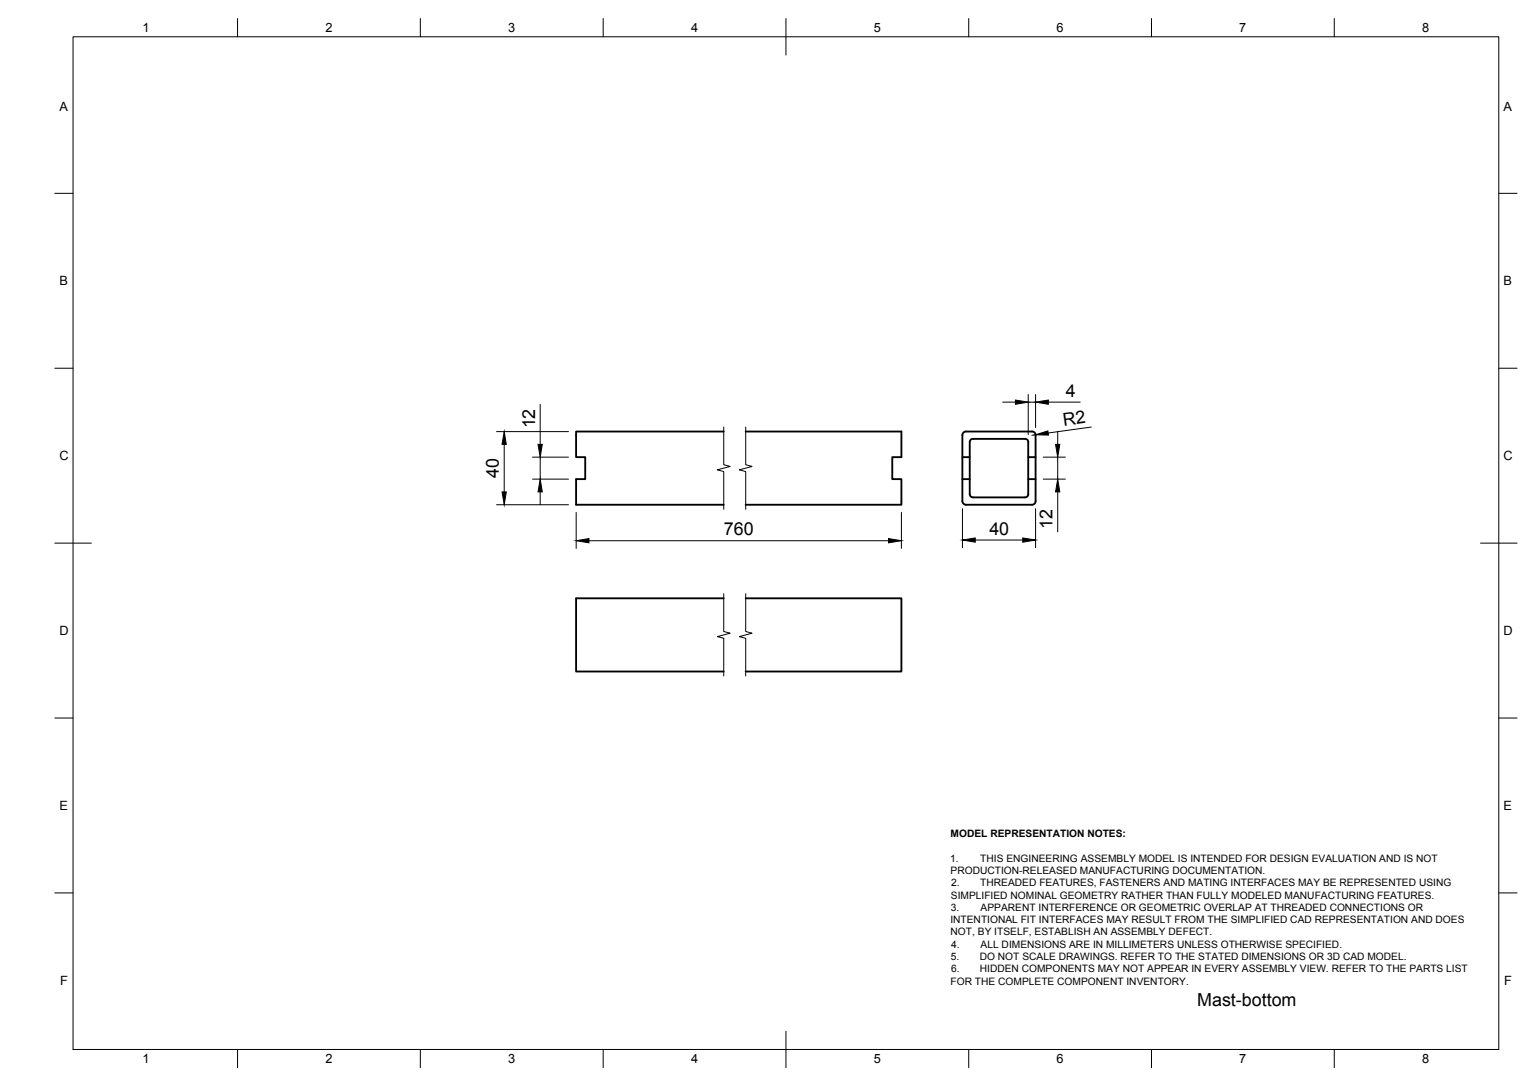
ISO-10303-21;
HEADER;
/* Generated by software containing ST-Developer
 * from STEP Tools, Inc. (www.steptools.com) 
 */

FILE_DESCRIPTION(
/* description */ (''),
/* implementation_level */ '2;1');

FILE_NAME(
/* name */ 'Mast-bottom.step',
/* time_stamp */ '2026-10-07T11:02:43-07:00',
/* author */ (''),
/* organization */ (''),
/* preprocessor_version */ 'ST-DEVELOPER v20.2',
/* originating_system */ 'Autodesk Translation Framework v15.15.0.0',
/* authorisation */ '');

FILE_SCHEMA (('AUTOMOTIVE_DESIGN { 1 0 10303 214 3 1 1 }'));
ENDSEC;

DATA;
#10=MECHANICAL_DESIGN_GEOMETRIC_PRESENTATION_REPRESENTATION('',(#66),#5505);
#52=SHAPE_REPRESENTATION_RELATIONSHIP('SRR','None',#5537,#59);
#59=ADVANCED_BREP_SHAPE_REPRESENTATION('',(#73),#5498);
#66=STYLED_ITEM('',(#5581),#73);
#73=MANIFOLD_SOLID_BREP('Body1',#3293);
#80=FACE_BOUND('',#416,.T.);
#81=FACE_BOUND('',#417,.T.);
#82=FACE_BOUND('',#428,.T.);
#83=FACE_BOUND('',#429,.T.);
#113=CYLINDRICAL_SURFACE('',#3399,2.);
#114=CYLINDRICAL_SURFACE('',#3401,2.);
#115=CYLINDRICAL_SURFACE('',#3404,2.);
#116=CYLINDRICAL_SURFACE('',#3406,2.);
#117=CYLINDRICAL_SURFACE('',#3414,1.8);
#118=CYLINDRICAL_SURFACE('',#3415,1.8);
#119=CYLINDRICAL_SURFACE('',#3417,1.8);
#120=CYLINDRICAL_SURFACE('',#3418,1.8);
#153=CIRCLE('',#3385,1.8);
#154=CIRCLE('',#3386,1.8);
#155=CIRCLE('',#3387,2.);
#156=CIRCLE('',#3388,2.);
#157=CIRCLE('',#3392,2.);
#158=CIRCLE('',#3393,2.);
#159=CIRCLE('',#3394,1.8);
#160=CIRCLE('',#3395,1.8);
#161=CIRCLE('',#3400,2.);
#162=CIRCLE('',#3402,2.);
#163=CIRCLE('',#3405,2.);
#164=CIRCLE('',#3407,2.);
#165=CIRCLE('',#3409,1.8);
#166=CIRCLE('',#3410,1.8);
#167=CIRCLE('',#3412,1.8);
#168=CIRCLE('',#3413,1.8);
#236=FACE_OUTER_BOUND('',#402,.T.);
#237=FACE_OUTER_BOUND('',#403,.T.);
#238=FACE_OUTER_BOUND('',#404,.T.);
#239=FACE_OUTER_BOUND('',#405,.T.);
#240=FACE_OUTER_BOUND('',#406,.T.);
#241=FACE_OUTER_BOUND('',#407,.T.);
#242=FACE_OUTER_BOUND('',#408,.T.);
#243=FACE_OUTER_BOUND('',#409,.T.);
#244=FACE_OUTER_BOUND('',#410,.T.);
#245=FACE_OUTER_BOUND('',#411,.T.);
#246=FACE_OUTER_BOUND('',#412,.T.);
#247=FACE_OUTER_BOUND('',#413,.T.);
#248=FACE_OUTER_BOUND('',#414,.T.);
#249=FACE_OUTER_BOUND('',#415,.T.);
#250=FACE_OUTER_BOUND('',#418,.T.);
#251=FACE_OUTER_BOUND('',#419,.T.);
#252=FACE_OUTER_BOUND('',#420,.T.);
#253=FACE_OUTER_BOUND('',#421,.T.);
#254=FACE_OUTER_BOUND('',#422,.T.);
#255=FACE_OUTER_BOUND('',#423,.T.);
#256=FACE_OUTER_BOUND('',#424,.T.);
#257=FACE_OUTER_BOUND('',#425,.T.);
#258=FACE_OUTER_BOUND('',#426,.T.);
#259=FACE_OUTER_BOUND('',#427,.T.);
#260=FACE_OUTER_BOUND('',#430,.T.);
#261=FACE_OUTER_BOUND('',#431,.T.);
#262=FACE_OUTER_BOUND('',#432,.T.);
#263=FACE_OUTER_BOUND('',#433,.T.);
#264=FACE_OUTER_BOUND('',#434,.T.);
#265=FACE_OUTER_BOUND('',#435,.T.);
#266=FACE_OUTER_BOUND('',#436,.T.);
#267=FACE_OUTER_BOUND('',#437,.T.);
#268=FACE_OUTER_BOUND('',#438,.T.);
#269=FACE_OUTER_BOUND('',#439,.T.);
#270=FACE_OUTER_BOUND('',#440,.T.);
#271=FACE_OUTER_BOUND('',#441,.T.);
#272=FACE_OUTER_BOUND('',#442,.T.);
#273=FACE_OUTER_BOUND('',#443,.T.);
#274=FACE_OUTER_BOUND('',#444,.T.);
#275=FACE_OUTER_BOUND('',#445,.T.);
#402=EDGE_LOOP('',(#2096,#2097,#2098,#2099));
#403=EDGE_LOOP('',(#2100,#2101,#2102,#2103));
#404=EDGE_LOOP('',(#2104,#2105,#2106,#2107));
#405=EDGE_LOOP('',(#2108,#2109,#2110,#2111));
#406=EDGE_LOOP('',(#2112,#2113,#2114,#2115,#2116,#2117,#2118,#2119,#2120,
#2121,#2122,#2123));
#407=EDGE_LOOP('',(#2124,#2125,#2126,#2127,#2128,#2129,#2130,#2131,#2132,
#2133,#2134,#2135));
#408=EDGE_LOOP('',(#2136,#2137,#2138,#2139,#2140,#2141,#2142,#2143,#2144,
#2145,#2146,#2147));
#409=EDGE_LOOP('',(#2148,#2149,#2150,#2151,#2152,#2153,#2154,#2155,#2156,
#2157,#2158,#2159));
#410=EDGE_LOOP('',(#2160,#2161,#2162,#2163,#2164,#2165,#2166,#2167,#2168,
#2169,#2170,#2171));
#411=EDGE_LOOP('',(#2172,#2173,#2174,#2175,#2176,#2177,#2178,#2179,#2180,
#2181,#2182,#2183));
#412=EDGE_LOOP('',(#2184,#2185,#2186,#2187));
#413=EDGE_LOOP('',(#2188,#2189,#2190,#2191));
#414=EDGE_LOOP('',(#2192,#2193,#2194,#2195));
#415=EDGE_LOOP('',(#2196,#2197,#2198,#2199));
#416=EDGE_LOOP('',(#2200,#2201,#2202,#2203));
#417=EDGE_LOOP('',(#2204,#2205,#2206,#2207));
#418=EDGE_LOOP('',(#2208,#2209,#2210,#2211));
#419=EDGE_LOOP('',(#2212,#2213,#2214,#2215));
#420=EDGE_LOOP('',(#2216,#2217,#2218,#2219,#2220,#2221,#2222,#2223,#2224,
#2225,#2226,#2227));
#421=EDGE_LOOP('',(#2228,#2229,#2230,#2231,#2232,#2233,#2234,#2235,#2236,
#2237,#2238,#2239));
#422=EDGE_LOOP('',(#2240,#2241,#2242,#2243));
#423=EDGE_LOOP('',(#2244,#2245,#2246,#2247));
#424=EDGE_LOOP('',(#2248,#2249,#2250,#2251));
#425=EDGE_LOOP('',(#2252,#2253,#2254,#2255));
#426=EDGE_LOOP('',(#2256,#2257,#2258,#2259));
#427=EDGE_LOOP('',(#2260,#2261,#2262,#2263));
#428=EDGE_LOOP('',(#2264,#2265,#2266,#2267));
#429=EDGE_LOOP('',(#2268,#2269,#2270,#2271));
#430=EDGE_LOOP('',(#2272,#2273,#2274,#2275));
#431=EDGE_LOOP('',(#2276,#2277,#2278,#2279));
#432=EDGE_LOOP('',(#2280,#2281,#2282,#2283));
#433=EDGE_LOOP('',(#2284,#2285,#2286,#2287));
#434=EDGE_LOOP('',(#2288,#2289,#2290,#2291));
#435=EDGE_LOOP('',(#2292,#2293,#2294,#2295));
#436=EDGE_LOOP('',(#2296,#2297,#2298,#2299));
#437=EDGE_LOOP('',(#2300,#2301,#2302,#2303));
#438=EDGE_LOOP('',(#2304,#2305,#2306,#2307));
#439=EDGE_LOOP('',(#2308,#2309,#2310,#2311));
#440=EDGE_LOOP('',(#2312,#2313,#2314,#2315));
#441=EDGE_LOOP('',(#2316,#2317,#2318,#2319));
#442=EDGE_LOOP('',(#2320,#2321,#2322,#2323));
#443=EDGE_LOOP('',(#2324,#2325,#2326,#2327));
#444=EDGE_LOOP('',(#2328,#2329,#2330,#2331));
#445=EDGE_LOOP('',(#2332,#2333,#2334,#2335));
#601=LINE('',#4554,#971);
#602=LINE('',#4556,#972);
#603=LINE('',#4558,#973);
#604=LINE('',#4559,#974);
#605=LINE('',#4562,#975);
#606=LINE('',#4564,#976);
#607=LINE('',#4565,#977);
#608=LINE('',#4568,#978);
#609=LINE('',#4570,#979);
#610=LINE('',#4571,#980);
#611=LINE('',#4573,#981);
#612=LINE('',#4574,#982);
#613=LINE('',#4578,#983);
#614=LINE('',#4580,#984);
#615=LINE('',#4582,#985);
#616=LINE('',#4586,#986);
#617=LINE('',#4590,#987);
#618=LINE('',#4592,#988);
#619=LINE('',#4594,#989);
#620=LINE('',#4598,#990);
#621=LINE('',#4603,#991);
#622=LINE('',#4605,#992);
#623=LINE('',#4606,#993);
#624=LINE('',#4608,#994);
#625=LINE('',#4610,#995);
#626=LINE('',#4612,#996);
#627=LINE('',#4614,#997);
#628=LINE('',#4616,#998);
#629=LINE('',#4618,#999);
#630=LINE('',#4620,#1000);
#631=LINE('',#4621,#1001);
#632=LINE('',#4625,#1002);
#633=LINE('',#4627,#1003);
#634=LINE('',#4629,#1004);
#635=LINE('',#4631,#1005);
#636=LINE('',#4633,#1006);
#637=LINE('',#4635,#1007);
#638=LINE('',#4637,#1008);
#639=LINE('',#4639,#1009);
#640=LINE('',#4640,#1010);
#641=LINE('',#4642,#1011);
#642=LINE('',#4643,#1012);
#643=LINE('',#4646,#1013);
#644=LINE('',#4648,#1014);
#645=LINE('',#4652,#1015);
#646=LINE('',#4656,#1016);
#647=LINE('',#4657,#1017);
#648=LINE('',#4661,#1018);
#649=LINE('',#4666,#1019);
#650=LINE('',#4668,#1020);
#651=LINE('',#4669,#1021);
#652=LINE('',#4671,#1022);
#653=LINE('',#4673,#1023);
#654=LINE('',#4675,#1024);
#655=LINE('',#4677,#1025);
#656=LINE('',#4678,#1026);
#657=LINE('',#4680,#1027);
#658=LINE('',#4681,#1028);
#659=LINE('',#4685,#1029);
#660=LINE('',#4687,#1030);
#661=LINE('',#4688,#1031);
#662=LINE('',#4690,#1032);
#663=LINE('',#4692,#1033);
#664=LINE('',#4694,#1034);
#665=LINE('',#4696,#1035);
#666=LINE('',#4697,#1036);
#667=LINE('',#4699,#1037);
#668=LINE('',#4700,#1038);
#669=LINE('',#4704,#1039);
#670=LINE('',#4705,#1040);
#671=LINE('',#4706,#1041);
#672=LINE('',#4711,#1042);
#673=LINE('',#4715,#1043);
#674=LINE('',#4716,#1044);
#675=LINE('',#4719,#1045);
#676=LINE('',#4721,#1046);
#677=LINE('',#4723,#1047);
#678=LINE('',#4724,#1048);
#679=LINE('',#4730,#1049);
#680=LINE('',#4731,#1050);
#681=LINE('',#4735,#1051);
#682=LINE('',#4738,#1052);
#683=LINE('',#4742,#1053);
#684=LINE('',#4744,#1054);
#685=LINE('',#4746,#1055);
#686=LINE('',#4748,#1056);
#687=LINE('',#4750,#1057);
#688=LINE('',#4753,#1058);
#689=LINE('',#4757,#1059);
#690=LINE('',#4759,#1060);
#691=LINE('',#4761,#1061);
#692=LINE('',#4762,#1062);
#693=LINE('',#4764,#1063);
#694=LINE('',#4766,#1064);
#695=LINE('',#4769,#1065);
#696=LINE('',#4771,#1066);
#697=LINE('',#4774,#1067);
#698=LINE('',#4776,#1068);
#699=LINE('',#4779,#1069);
#700=LINE('',#4781,#1070);
#701=LINE('',#4784,#1071);
#702=LINE('',#4785,#1072);
#703=LINE('',#4787,#1073);
#704=LINE('',#4789,#1074);
#971=VECTOR('',#3651,1000.);
#972=VECTOR('',#3652,1000.);
#973=VECTOR('',#3653,1000.);
#974=VECTOR('',#3654,1000.);
#975=VECTOR('',#3657,1000.);
#976=VECTOR('',#3658,1000.);
#977=VECTOR('',#3659,1000.);
#978=VECTOR('',#3662,1000.);
#979=VECTOR('',#3663,1000.);
#980=VECTOR('',#3664,1000.);
#981=VECTOR('',#3667,1000.);
#982=VECTOR('',#3668,1000.);
#983=VECTOR('',#3671,1000.);
#984=VECTOR('',#3672,1000.);
#985=VECTOR('',#3673,1000.);
#986=VECTOR('',#3676,1000.);
#987=VECTOR('',#3679,1000.);
#988=VECTOR('',#3680,1000.);
#989=VECTOR('',#3681,1000.);
#990=VECTOR('',#3684,1000.);
#991=VECTOR('',#3689,1000.);
#992=VECTOR('',#3690,1000.);
#993=VECTOR('',#3691,1000.);
#994=VECTOR('',#3692,1000.);
#995=VECTOR('',#3693,1000.);
#996=VECTOR('',#3694,1000.);
#997=VECTOR('',#3695,1000.);
#998=VECTOR('',#3696,1000.);
#999=VECTOR('',#3697,1000.);
#1000=VECTOR('',#3698,1000.);
#1001=VECTOR('',#3699,1000.);
#1002=VECTOR('',#3702,1000.);
#1003=VECTOR('',#3703,1000.);
#1004=VECTOR('',#3704,1000.);
#1005=VECTOR('',#3705,1000.);
#1006=VECTOR('',#3706,1000.);
#1007=VECTOR('',#3707,1000.);
#1008=VECTOR('',#3708,1000.);
#1009=VECTOR('',#3709,1000.);
#1010=VECTOR('',#3710,1000.);
#1011=VECTOR('',#3711,1000.);
#1012=VECTOR('',#3712,1000.);
#1013=VECTOR('',#3715,1000.);
#1014=VECTOR('',#3716,1000.);
#1015=VECTOR('',#3719,1000.);
#1016=VECTOR('',#3722,1000.);
#1017=VECTOR('',#3723,1000.);
#1018=VECTOR('',#3726,1000.);
#1019=VECTOR('',#3731,1000.);
#1020=VECTOR('',#3732,1000.);
#1021=VECTOR('',#3733,1000.);
#1022=VECTOR('',#3734,1000.);
#1023=VECTOR('',#3735,1000.);
#1024=VECTOR('',#3736,1000.);
#1025=VECTOR('',#3737,1000.);
#1026=VECTOR('',#3738,1000.);
#1027=VECTOR('',#3739,1000.);
#1028=VECTOR('',#3740,1000.);
#1029=VECTOR('',#3743,1000.);
#1030=VECTOR('',#3744,1000.);
#1031=VECTOR('',#3745,1000.);
#1032=VECTOR('',#3746,1000.);
#1033=VECTOR('',#3747,1000.);
#1034=VECTOR('',#3748,1000.);
#1035=VECTOR('',#3749,1000.);
#1036=VECTOR('',#3750,1000.);
#1037=VECTOR('',#3751,1000.);
#1038=VECTOR('',#3752,1000.);
#1039=VECTOR('',#3755,1000.);
#1040=VECTOR('',#3756,1000.);
#1041=VECTOR('',#3757,1000.);
#1042=VECTOR('',#3764,1000.);
#1043=VECTOR('',#3769,1000.);
#1044=VECTOR('',#3770,1000.);
#1045=VECTOR('',#3771,1000.);
#1046=VECTOR('',#3772,1000.);
#1047=VECTOR('',#3773,1000.);
#1048=VECTOR('',#3774,1000.);
#1049=VECTOR('',#3785,1000.);
#1050=VECTOR('',#3786,1000.);
#1051=VECTOR('',#3789,1000.);
#1052=VECTOR('',#3794,1000.);
#1053=VECTOR('',#3797,1000.);
#1054=VECTOR('',#3800,1000.);
#1055=VECTOR('',#3803,1000.);
#1056=VECTOR('',#3806,1000.);
#1057=VECTOR('',#3809,1000.);
#1058=VECTOR('',#3814,1000.);
#1059=VECTOR('',#3817,1000.);
#1060=VECTOR('',#3818,1000.);
#1061=VECTOR('',#3819,1000.);
#1062=VECTOR('',#3820,1000.);
#1063=VECTOR('',#3823,1000.);
#1064=VECTOR('',#3826,1000.);
#1065=VECTOR('',#3831,1000.);
#1066=VECTOR('',#3834,1000.);
#1067=VECTOR('',#3839,1000.);
#1068=VECTOR('',#3842,1000.);
#1069=VECTOR('',#3847,1000.);
#1070=VECTOR('',#3850,1000.);
#1071=VECTOR('',#3855,1000.);
#1072=VECTOR('',#3856,1000.);
#1073=VECTOR('',#3859,1000.);
#1074=VECTOR('',#3862,1000.);
#1341=VERTEX_POINT('',#4552);
#1342=VERTEX_POINT('',#4553);
#1343=VERTEX_POINT('',#4555);
#1344=VERTEX_POINT('',#4557);
#1345=VERTEX_POINT('',#4561);
#1346=VERTEX_POINT('',#4563);
#1347=VERTEX_POINT('',#4567);
#1348=VERTEX_POINT('',#4569);
#1349=VERTEX_POINT('',#4576);
#1350=VERTEX_POINT('',#4577);
#1351=VERTEX_POINT('',#4579);
#1352=VERTEX_POINT('',#4581);
#1353=VERTEX_POINT('',#4583);
#1354=VERTEX_POINT('',#4585);
#1355=VERTEX_POINT('',#4587);
#1356=VERTEX_POINT('',#4589);
#1357=VERTEX_POINT('',#4591);
#1358=VERTEX_POINT('',#4593);
#1359=VERTEX_POINT('',#4595);
#1360=VERTEX_POINT('',#4597);
#1361=VERTEX_POINT('',#4601);
#1362=VERTEX_POINT('',#4602);
#1363=VERTEX_POINT('',#4604);
#1364=VERTEX_POINT('',#4607);
#1365=VERTEX_POINT('',#4609);
#1366=VERTEX_POINT('',#4611);
#1367=VERTEX_POINT('',#4613);
#1368=VERTEX_POINT('',#4615);
#1369=VERTEX_POINT('',#4617);
#1370=VERTEX_POINT('',#4619);
#1371=VERTEX_POINT('',#4623);
#1372=VERTEX_POINT('',#4624);
#1373=VERTEX_POINT('',#4626);
#1374=VERTEX_POINT('',#4628);
#1375=VERTEX_POINT('',#4630);
#1376=VERTEX_POINT('',#4632);
#1377=VERTEX_POINT('',#4634);
#1378=VERTEX_POINT('',#4636);
#1379=VERTEX_POINT('',#4638);
#1380=VERTEX_POINT('',#4641);
#1381=VERTEX_POINT('',#4645);
#1382=VERTEX_POINT('',#4647);
#1383=VERTEX_POINT('',#4649);
#1384=VERTEX_POINT('',#4651);
#1385=VERTEX_POINT('',#4653);
#1386=VERTEX_POINT('',#4655);
#1387=VERTEX_POINT('',#4658);
#1388=VERTEX_POINT('',#4660);
#1389=VERTEX_POINT('',#4664);
#1390=VERTEX_POINT('',#4665);
#1391=VERTEX_POINT('',#4667);
#1392=VERTEX_POINT('',#4670);
#1393=VERTEX_POINT('',#4672);
#1394=VERTEX_POINT('',#4674);
#1395=VERTEX_POINT('',#4676);
#1396=VERTEX_POINT('',#4679);
#1397=VERTEX_POINT('',#4683);
#1398=VERTEX_POINT('',#4684);
#1399=VERTEX_POINT('',#4686);
#1400=VERTEX_POINT('',#4689);
#1401=VERTEX_POINT('',#4691);
#1402=VERTEX_POINT('',#4693);
#1403=VERTEX_POINT('',#4695);
#1404=VERTEX_POINT('',#4698);
#1405=VERTEX_POINT('',#4702);
#1406=VERTEX_POINT('',#4703);
#1407=VERTEX_POINT('',#4710);
#1408=VERTEX_POINT('',#4714);
#1409=VERTEX_POINT('',#4717);
#1410=VERTEX_POINT('',#4718);
#1411=VERTEX_POINT('',#4720);
#1412=VERTEX_POINT('',#4722);
#1413=VERTEX_POINT('',#4732);
#1414=VERTEX_POINT('',#4734);
#1415=VERTEX_POINT('',#4739);
#1416=VERTEX_POINT('',#4741);
#1417=VERTEX_POINT('',#4755);
#1418=VERTEX_POINT('',#4756);
#1419=VERTEX_POINT('',#4758);
#1420=VERTEX_POINT('',#4760);
#1643=EDGE_CURVE('',#1341,#1342,#601,.T.);
#1644=EDGE_CURVE('',#1341,#1343,#602,.T.);
#1645=EDGE_CURVE('',#1343,#1344,#603,.T.);
#1646=EDGE_CURVE('',#1344,#1342,#604,.T.);
#1647=EDGE_CURVE('',#1343,#1345,#605,.T.);
#1648=EDGE_CURVE('',#1345,#1346,#606,.T.);
#1649=EDGE_CURVE('',#1346,#1344,#607,.T.);
#1650=EDGE_CURVE('',#1347,#1345,#608,.T.);
#1651=EDGE_CURVE('',#1347,#1348,#609,.T.);
#1652=EDGE_CURVE('',#1346,#1348,#610,.T.);
#1653=EDGE_CURVE('',#1341,#1347,#611,.T.);
#1654=EDGE_CURVE('',#1348,#1342,#612,.T.);
#1655=EDGE_CURVE('',#1349,#1350,#613,.T.);
#1656=EDGE_CURVE('',#1350,#1351,#614,.T.);
#1657=EDGE_CURVE('',#1351,#1352,#615,.T.);
#1658=EDGE_CURVE('',#1353,#1352,#153,.T.);
#1659=EDGE_CURVE('',#1353,#1354,#616,.T.);
#1660=EDGE_CURVE('',#1355,#1354,#154,.T.);
#1661=EDGE_CURVE('',#1356,#1355,#617,.T.);
#1662=EDGE_CURVE('',#1356,#1357,#618,.T.);
#1663=EDGE_CURVE('',#1357,#1358,#619,.T.);
#1664=EDGE_CURVE('',#1358,#1359,#155,.T.);
#1665=EDGE_CURVE('',#1359,#1360,#620,.T.);
#1666=EDGE_CURVE('',#1360,#1349,#156,.T.);
#1667=EDGE_CURVE('',#1361,#1362,#621,.T.);
#1668=EDGE_CURVE('',#1363,#1361,#622,.T.);
#1669=EDGE_CURVE('',#1363,#1356,#623,.T.);
#1670=EDGE_CURVE('',#1364,#1355,#624,.T.);
#1671=EDGE_CURVE('',#1365,#1364,#625,.F.);
#1672=EDGE_CURVE('',#1366,#1365,#626,.T.);
#1673=EDGE_CURVE('',#1366,#1367,#627,.T.);
#1674=EDGE_CURVE('',#1367,#1368,#628,.T.);
#1675=EDGE_CURVE('',#1369,#1368,#629,.F.);
#1676=EDGE_CURVE('',#1369,#1370,#630,.T.);
#1677=EDGE_CURVE('',#1370,#1362,#631,.T.);
#1678=EDGE_CURVE('',#1371,#1372,#632,.T.);
#1679=EDGE_CURVE('',#1373,#1371,#633,.T.);
#1680=EDGE_CURVE('',#1374,#1373,#634,.T.);
#1681=EDGE_CURVE('',#1374,#1375,#635,.F.);
#1682=EDGE_CURVE('',#1375,#1376,#636,.T.);
#1683=EDGE_CURVE('',#1376,#1377,#637,.T.);
#1684=EDGE_CURVE('',#1378,#1377,#638,.T.);
#1685=EDGE_CURVE('',#1378,#1379,#639,.F.);
#1686=EDGE_CURVE('',#1379,#1352,#640,.T.);
#1687=EDGE_CURVE('',#1351,#1380,#641,.T.);
#1688=EDGE_CURVE('',#1372,#1380,#642,.T.);
#1689=EDGE_CURVE('',#1381,#1368,#643,.F.);
#1690=EDGE_CURVE('',#1382,#1381,#644,.F.);
#1691=EDGE_CURVE('',#1383,#1382,#157,.F.);
#1692=EDGE_CURVE('',#1384,#1383,#645,.F.);
#1693=EDGE_CURVE('',#1385,#1384,#158,.F.);
#1694=EDGE_CURVE('',#1386,#1385,#646,.F.);
#1695=EDGE_CURVE('',#1375,#1386,#647,.F.);
#1696=EDGE_CURVE('',#1374,#1387,#159,.F.);
#1697=EDGE_CURVE('',#1387,#1388,#648,.F.);
#1698=EDGE_CURVE('',#1388,#1369,#160,.F.);
#1699=EDGE_CURVE('',#1389,#1390,#649,.T.);
#1700=EDGE_CURVE('',#1391,#1389,#650,.T.);
#1701=EDGE_CURVE('',#1382,#1391,#651,.T.);
#1702=EDGE_CURVE('',#1381,#1392,#652,.T.);
#1703=EDGE_CURVE('',#1392,#1393,#653,.T.);
#1704=EDGE_CURVE('',#1394,#1393,#654,.T.);
#1705=EDGE_CURVE('',#1394,#1395,#655,.F.);
#1706=EDGE_CURVE('',#1395,#1358,#656,.T.);
#1707=EDGE_CURVE('',#1357,#1396,#657,.T.);
#1708=EDGE_CURVE('',#1390,#1396,#658,.T.);
#1709=EDGE_CURVE('',#1397,#1398,#659,.T.);
#1710=EDGE_CURVE('',#1399,#1397,#660,.T.);
#1711=EDGE_CURVE('',#1399,#1350,#661,.T.);
#1712=EDGE_CURVE('',#1400,#1349,#662,.T.);
#1713=EDGE_CURVE('',#1400,#1401,#663,.F.);
#1714=EDGE_CURVE('',#1402,#1401,#664,.T.);
#1715=EDGE_CURVE('',#1402,#1403,#665,.T.);
#1716=EDGE_CURVE('',#1403,#1386,#666,.T.);
#1717=EDGE_CURVE('',#1385,#1404,#667,.T.);
#1718=EDGE_CURVE('',#1398,#1404,#668,.T.);
#1719=EDGE_CURVE('',#1405,#1406,#669,.T.);
#1720=EDGE_CURVE('',#1384,#1405,#670,.T.);
#1721=EDGE_CURVE('',#1383,#1406,#671,.T.);
#1722=EDGE_CURVE('',#1404,#1405,#161,.T.);
#1723=EDGE_CURVE('',#1407,#1360,#672,.T.);
#1724=EDGE_CURVE('',#1407,#1400,#162,.F.);
#1725=EDGE_CURVE('',#1408,#1359,#673,.T.);
#1726=EDGE_CURVE('',#1408,#1407,#674,.F.);
#1727=EDGE_CURVE('',#1409,#1410,#675,.T.);
#1728=EDGE_CURVE('',#1409,#1411,#676,.T.);
#1729=EDGE_CURVE('',#1411,#1412,#677,.T.);
#1730=EDGE_CURVE('',#1410,#1412,#678,.T.);
#1731=EDGE_CURVE('',#1395,#1408,#163,.F.);
#1732=EDGE_CURVE('',#1406,#1391,#164,.T.);
#1733=EDGE_CURVE('',#1398,#1371,#679,.T.);
#1734=EDGE_CURVE('',#1362,#1389,#680,.T.);
#1735=EDGE_CURVE('',#1413,#1370,#165,.T.);
#1736=EDGE_CURVE('',#1414,#1413,#681,.T.);
#1737=EDGE_CURVE('',#1373,#1414,#166,.T.);
#1738=EDGE_CURVE('',#1394,#1365,#682,.F.);
#1739=EDGE_CURVE('',#1364,#1415,#167,.F.);
#1740=EDGE_CURVE('',#1416,#1415,#683,.F.);
#1741=EDGE_CURVE('',#1416,#1379,#168,.F.);
#1742=EDGE_CURVE('',#1378,#1401,#684,.F.);
#1743=EDGE_CURVE('',#1416,#1353,#685,.T.);
#1744=EDGE_CURVE('',#1387,#1414,#686,.T.);
#1745=EDGE_CURVE('',#1388,#1413,#687,.T.);
#1746=EDGE_CURVE('',#1415,#1354,#688,.T.);
#1747=EDGE_CURVE('',#1417,#1418,#689,.T.);
#1748=EDGE_CURVE('',#1419,#1417,#690,.T.);
#1749=EDGE_CURVE('',#1419,#1420,#691,.T.);
#1750=EDGE_CURVE('',#1420,#1418,#692,.T.);
#1751=EDGE_CURVE('',#1377,#1402,#693,.T.);
#1752=EDGE_CURVE('',#1376,#1403,#694,.T.);
#1753=EDGE_CURVE('',#1392,#1367,#695,.T.);
#1754=EDGE_CURVE('',#1393,#1366,#696,.T.);
#1755=EDGE_CURVE('',#1390,#1361,#697,.T.);
#1756=EDGE_CURVE('',#1396,#1363,#698,.T.);
#1757=EDGE_CURVE('',#1372,#1397,#699,.T.);
#1758=EDGE_CURVE('',#1380,#1399,#700,.T.);
#1759=EDGE_CURVE('',#1418,#1409,#701,.T.);
#1760=EDGE_CURVE('',#1417,#1410,#702,.T.);
#1761=EDGE_CURVE('',#1419,#1412,#703,.T.);
#1762=EDGE_CURVE('',#1420,#1411,#704,.T.);
#2096=ORIENTED_EDGE('',*,*,#1643,.F.);
#2097=ORIENTED_EDGE('',*,*,#1644,.T.);
#2098=ORIENTED_EDGE('',*,*,#1645,.T.);
#2099=ORIENTED_EDGE('',*,*,#1646,.T.);
#2100=ORIENTED_EDGE('',*,*,#1645,.F.);
#2101=ORIENTED_EDGE('',*,*,#1647,.T.);
#2102=ORIENTED_EDGE('',*,*,#1648,.T.);
#2103=ORIENTED_EDGE('',*,*,#1649,.T.);
#2104=ORIENTED_EDGE('',*,*,#1650,.F.);
#2105=ORIENTED_EDGE('',*,*,#1651,.T.);
#2106=ORIENTED_EDGE('',*,*,#1652,.F.);
#2107=ORIENTED_EDGE('',*,*,#1648,.F.);
#2108=ORIENTED_EDGE('',*,*,#1653,.F.);
#2109=ORIENTED_EDGE('',*,*,#1643,.T.);
#2110=ORIENTED_EDGE('',*,*,#1654,.F.);
#2111=ORIENTED_EDGE('',*,*,#1651,.F.);
#2112=ORIENTED_EDGE('',*,*,#1655,.T.);
#2113=ORIENTED_EDGE('',*,*,#1656,.T.);
#2114=ORIENTED_EDGE('',*,*,#1657,.T.);
#2115=ORIENTED_EDGE('',*,*,#1658,.F.);
#2116=ORIENTED_EDGE('',*,*,#1659,.T.);
#2117=ORIENTED_EDGE('',*,*,#1660,.F.);
#2118=ORIENTED_EDGE('',*,*,#1661,.F.);
#2119=ORIENTED_EDGE('',*,*,#1662,.T.);
#2120=ORIENTED_EDGE('',*,*,#1663,.T.);
#2121=ORIENTED_EDGE('',*,*,#1664,.T.);
#2122=ORIENTED_EDGE('',*,*,#1665,.T.);
#2123=ORIENTED_EDGE('',*,*,#1666,.T.);
#2124=ORIENTED_EDGE('',*,*,#1667,.F.);
#2125=ORIENTED_EDGE('',*,*,#1668,.F.);
#2126=ORIENTED_EDGE('',*,*,#1669,.T.);
#2127=ORIENTED_EDGE('',*,*,#1661,.T.);
#2128=ORIENTED_EDGE('',*,*,#1670,.F.);
#2129=ORIENTED_EDGE('',*,*,#1671,.F.);
#2130=ORIENTED_EDGE('',*,*,#1672,.F.);
#2131=ORIENTED_EDGE('',*,*,#1673,.T.);
#2132=ORIENTED_EDGE('',*,*,#1674,.T.);
#2133=ORIENTED_EDGE('',*,*,#1675,.F.);
#2134=ORIENTED_EDGE('',*,*,#1676,.T.);
#2135=ORIENTED_EDGE('',*,*,#1677,.T.);
#2136=ORIENTED_EDGE('',*,*,#1678,.F.);
#2137=ORIENTED_EDGE('',*,*,#1679,.F.);
#2138=ORIENTED_EDGE('',*,*,#1680,.F.);
#2139=ORIENTED_EDGE('',*,*,#1681,.T.);
#2140=ORIENTED_EDGE('',*,*,#1682,.T.);
#2141=ORIENTED_EDGE('',*,*,#1683,.T.);
#2142=ORIENTED_EDGE('',*,*,#1684,.F.);
#2143=ORIENTED_EDGE('',*,*,#1685,.T.);
#2144=ORIENTED_EDGE('',*,*,#1686,.T.);
#2145=ORIENTED_EDGE('',*,*,#1657,.F.);
#2146=ORIENTED_EDGE('',*,*,#1687,.T.);
#2147=ORIENTED_EDGE('',*,*,#1688,.F.);
#2148=ORIENTED_EDGE('',*,*,#1689,.F.);
#2149=ORIENTED_EDGE('',*,*,#1690,.F.);
#2150=ORIENTED_EDGE('',*,*,#1691,.F.);
#2151=ORIENTED_EDGE('',*,*,#1692,.F.);
#2152=ORIENTED_EDGE('',*,*,#1693,.F.);
#2153=ORIENTED_EDGE('',*,*,#1694,.F.);
#2154=ORIENTED_EDGE('',*,*,#1695,.F.);
#2155=ORIENTED_EDGE('',*,*,#1681,.F.);
#2156=ORIENTED_EDGE('',*,*,#1696,.T.);
#2157=ORIENTED_EDGE('',*,*,#1697,.T.);
#2158=ORIENTED_EDGE('',*,*,#1698,.T.);
#2159=ORIENTED_EDGE('',*,*,#1675,.T.);
#2160=ORIENTED_EDGE('',*,*,#1699,.F.);
#2161=ORIENTED_EDGE('',*,*,#1700,.F.);
#2162=ORIENTED_EDGE('',*,*,#1701,.F.);
#2163=ORIENTED_EDGE('',*,*,#1690,.T.);
#2164=ORIENTED_EDGE('',*,*,#1702,.T.);
#2165=ORIENTED_EDGE('',*,*,#1703,.T.);
#2166=ORIENTED_EDGE('',*,*,#1704,.F.);
#2167=ORIENTED_EDGE('',*,*,#1705,.T.);
#2168=ORIENTED_EDGE('',*,*,#1706,.T.);
#2169=ORIENTED_EDGE('',*,*,#1663,.F.);
#2170=ORIENTED_EDGE('',*,*,#1707,.T.);
#2171=ORIENTED_EDGE('',*,*,#1708,.F.);
#2172=ORIENTED_EDGE('',*,*,#1709,.F.);
#2173=ORIENTED_EDGE('',*,*,#1710,.F.);
#2174=ORIENTED_EDGE('',*,*,#1711,.T.);
#2175=ORIENTED_EDGE('',*,*,#1655,.F.);
#2176=ORIENTED_EDGE('',*,*,#1712,.F.);
#2177=ORIENTED_EDGE('',*,*,#1713,.T.);
#2178=ORIENTED_EDGE('',*,*,#1714,.F.);
#2179=ORIENTED_EDGE('',*,*,#1715,.T.);
#2180=ORIENTED_EDGE('',*,*,#1716,.T.);
#2181=ORIENTED_EDGE('',*,*,#1694,.T.);
#2182=ORIENTED_EDGE('',*,*,#1717,.T.);
#2183=ORIENTED_EDGE('',*,*,#1718,.F.);
#2184=ORIENTED_EDGE('',*,*,#1719,.F.);
#2185=ORIENTED_EDGE('',*,*,#1720,.F.);
#2186=ORIENTED_EDGE('',*,*,#1692,.T.);
#2187=ORIENTED_EDGE('',*,*,#1721,.T.);
#2188=ORIENTED_EDGE('',*,*,#1720,.T.);
#2189=ORIENTED_EDGE('',*,*,#1722,.F.);
#2190=ORIENTED_EDGE('',*,*,#1717,.F.);
#2191=ORIENTED_EDGE('',*,*,#1693,.T.);
#2192=ORIENTED_EDGE('',*,*,#1712,.T.);
#2193=ORIENTED_EDGE('',*,*,#1666,.F.);
#2194=ORIENTED_EDGE('',*,*,#1723,.F.);
#2195=ORIENTED_EDGE('',*,*,#1724,.T.);
#2196=ORIENTED_EDGE('',*,*,#1723,.T.);
#2197=ORIENTED_EDGE('',*,*,#1665,.F.);
#2198=ORIENTED_EDGE('',*,*,#1725,.F.);
#2199=ORIENTED_EDGE('',*,*,#1726,.T.);
#2200=ORIENTED_EDGE('',*,*,#1652,.T.);
#2201=ORIENTED_EDGE('',*,*,#1654,.T.);
#2202=ORIENTED_EDGE('',*,*,#1646,.F.);
#2203=ORIENTED_EDGE('',*,*,#1649,.F.);
#2204=ORIENTED_EDGE('',*,*,#1727,.F.);
#2205=ORIENTED_EDGE('',*,*,#1728,.T.);
#2206=ORIENTED_EDGE('',*,*,#1729,.T.);
#2207=ORIENTED_EDGE('',*,*,#1730,.F.);
#2208=ORIENTED_EDGE('',*,*,#1725,.T.);
#2209=ORIENTED_EDGE('',*,*,#1664,.F.);
#2210=ORIENTED_EDGE('',*,*,#1706,.F.);
#2211=ORIENTED_EDGE('',*,*,#1731,.T.);
#2212=ORIENTED_EDGE('',*,*,#1701,.T.);
#2213=ORIENTED_EDGE('',*,*,#1732,.F.);
#2214=ORIENTED_EDGE('',*,*,#1721,.F.);
#2215=ORIENTED_EDGE('',*,*,#1691,.T.);
#2216=ORIENTED_EDGE('',*,*,#1733,.F.);
#2217=ORIENTED_EDGE('',*,*,#1718,.T.);
#2218=ORIENTED_EDGE('',*,*,#1722,.T.);
#2219=ORIENTED_EDGE('',*,*,#1719,.T.);
#2220=ORIENTED_EDGE('',*,*,#1732,.T.);
#2221=ORIENTED_EDGE('',*,*,#1700,.T.);
#2222=ORIENTED_EDGE('',*,*,#1734,.F.);
#2223=ORIENTED_EDGE('',*,*,#1677,.F.);
#2224=ORIENTED_EDGE('',*,*,#1735,.F.);
#2225=ORIENTED_EDGE('',*,*,#1736,.F.);
#2226=ORIENTED_EDGE('',*,*,#1737,.F.);
#2227=ORIENTED_EDGE('',*,*,#1679,.T.);
#2228=ORIENTED_EDGE('',*,*,#1705,.F.);
#2229=ORIENTED_EDGE('',*,*,#1738,.T.);
#2230=ORIENTED_EDGE('',*,*,#1671,.T.);
#2231=ORIENTED_EDGE('',*,*,#1739,.T.);
#2232=ORIENTED_EDGE('',*,*,#1740,.F.);
#2233=ORIENTED_EDGE('',*,*,#1741,.T.);
#2234=ORIENTED_EDGE('',*,*,#1685,.F.);
#2235=ORIENTED_EDGE('',*,*,#1742,.T.);
#2236=ORIENTED_EDGE('',*,*,#1713,.F.);
#2237=ORIENTED_EDGE('',*,*,#1724,.F.);
#2238=ORIENTED_EDGE('',*,*,#1726,.F.);
#2239=ORIENTED_EDGE('',*,*,#1731,.F.);
#2240=ORIENTED_EDGE('',*,*,#1658,.T.);
#2241=ORIENTED_EDGE('',*,*,#1686,.F.);
#2242=ORIENTED_EDGE('',*,*,#1741,.F.);
#2243=ORIENTED_EDGE('',*,*,#1743,.T.);
#2244=ORIENTED_EDGE('',*,*,#1680,.T.);
#2245=ORIENTED_EDGE('',*,*,#1737,.T.);
#2246=ORIENTED_EDGE('',*,*,#1744,.F.);
#2247=ORIENTED_EDGE('',*,*,#1696,.F.);
#2248=ORIENTED_EDGE('',*,*,#1744,.T.);
#2249=ORIENTED_EDGE('',*,*,#1736,.T.);
#2250=ORIENTED_EDGE('',*,*,#1745,.F.);
#2251=ORIENTED_EDGE('',*,*,#1697,.F.);
#2252=ORIENTED_EDGE('',*,*,#1745,.T.);
#2253=ORIENTED_EDGE('',*,*,#1735,.T.);
#2254=ORIENTED_EDGE('',*,*,#1676,.F.);
#2255=ORIENTED_EDGE('',*,*,#1698,.F.);
#2256=ORIENTED_EDGE('',*,*,#1670,.T.);
#2257=ORIENTED_EDGE('',*,*,#1660,.T.);
#2258=ORIENTED_EDGE('',*,*,#1746,.F.);
#2259=ORIENTED_EDGE('',*,*,#1739,.F.);
#2260=ORIENTED_EDGE('',*,*,#1746,.T.);
#2261=ORIENTED_EDGE('',*,*,#1659,.F.);
#2262=ORIENTED_EDGE('',*,*,#1743,.F.);
#2263=ORIENTED_EDGE('',*,*,#1740,.T.);
#2264=ORIENTED_EDGE('',*,*,#1650,.T.);
#2265=ORIENTED_EDGE('',*,*,#1647,.F.);
#2266=ORIENTED_EDGE('',*,*,#1644,.F.);
#2267=ORIENTED_EDGE('',*,*,#1653,.T.);
#2268=ORIENTED_EDGE('',*,*,#1747,.F.);
#2269=ORIENTED_EDGE('',*,*,#1748,.F.);
#2270=ORIENTED_EDGE('',*,*,#1749,.T.);
#2271=ORIENTED_EDGE('',*,*,#1750,.T.);
#2272=ORIENTED_EDGE('',*,*,#1684,.T.);
#2273=ORIENTED_EDGE('',*,*,#1751,.T.);
#2274=ORIENTED_EDGE('',*,*,#1714,.T.);
#2275=ORIENTED_EDGE('',*,*,#1742,.F.);
#2276=ORIENTED_EDGE('',*,*,#1752,.T.);
#2277=ORIENTED_EDGE('',*,*,#1715,.F.);
#2278=ORIENTED_EDGE('',*,*,#1751,.F.);
#2279=ORIENTED_EDGE('',*,*,#1683,.F.);
#2280=ORIENTED_EDGE('',*,*,#1695,.T.);
#2281=ORIENTED_EDGE('',*,*,#1716,.F.);
#2282=ORIENTED_EDGE('',*,*,#1752,.F.);
#2283=ORIENTED_EDGE('',*,*,#1682,.F.);
#2284=ORIENTED_EDGE('',*,*,#1753,.F.);
#2285=ORIENTED_EDGE('',*,*,#1702,.F.);
#2286=ORIENTED_EDGE('',*,*,#1689,.T.);
#2287=ORIENTED_EDGE('',*,*,#1674,.F.);
#2288=ORIENTED_EDGE('',*,*,#1754,.F.);
#2289=ORIENTED_EDGE('',*,*,#1703,.F.);
#2290=ORIENTED_EDGE('',*,*,#1753,.T.);
#2291=ORIENTED_EDGE('',*,*,#1673,.F.);
#2292=ORIENTED_EDGE('',*,*,#1672,.T.);
#2293=ORIENTED_EDGE('',*,*,#1738,.F.);
#2294=ORIENTED_EDGE('',*,*,#1704,.T.);
#2295=ORIENTED_EDGE('',*,*,#1754,.T.);
#2296=ORIENTED_EDGE('',*,*,#1667,.T.);
#2297=ORIENTED_EDGE('',*,*,#1734,.T.);
#2298=ORIENTED_EDGE('',*,*,#1699,.T.);
#2299=ORIENTED_EDGE('',*,*,#1755,.T.);
#2300=ORIENTED_EDGE('',*,*,#1756,.F.);
#2301=ORIENTED_EDGE('',*,*,#1707,.F.);
#2302=ORIENTED_EDGE('',*,*,#1662,.F.);
#2303=ORIENTED_EDGE('',*,*,#1669,.F.);
#2304=ORIENTED_EDGE('',*,*,#1668,.T.);
#2305=ORIENTED_EDGE('',*,*,#1755,.F.);
#2306=ORIENTED_EDGE('',*,*,#1708,.T.);
#2307=ORIENTED_EDGE('',*,*,#1756,.T.);
#2308=ORIENTED_EDGE('',*,*,#1678,.T.);
#2309=ORIENTED_EDGE('',*,*,#1757,.T.);
#2310=ORIENTED_EDGE('',*,*,#1709,.T.);
#2311=ORIENTED_EDGE('',*,*,#1733,.T.);
#2312=ORIENTED_EDGE('',*,*,#1656,.F.);
#2313=ORIENTED_EDGE('',*,*,#1711,.F.);
#2314=ORIENTED_EDGE('',*,*,#1758,.F.);
#2315=ORIENTED_EDGE('',*,*,#1687,.F.);
#2316=ORIENTED_EDGE('',*,*,#1688,.T.);
#2317=ORIENTED_EDGE('',*,*,#1758,.T.);
#2318=ORIENTED_EDGE('',*,*,#1710,.T.);
#2319=ORIENTED_EDGE('',*,*,#1757,.F.);
#2320=ORIENTED_EDGE('',*,*,#1747,.T.);
#2321=ORIENTED_EDGE('',*,*,#1759,.T.);
#2322=ORIENTED_EDGE('',*,*,#1727,.T.);
#2323=ORIENTED_EDGE('',*,*,#1760,.F.);
#2324=ORIENTED_EDGE('',*,*,#1748,.T.);
#2325=ORIENTED_EDGE('',*,*,#1760,.T.);
#2326=ORIENTED_EDGE('',*,*,#1730,.T.);
#2327=ORIENTED_EDGE('',*,*,#1761,.F.);
#2328=ORIENTED_EDGE('',*,*,#1761,.T.);
#2329=ORIENTED_EDGE('',*,*,#1729,.F.);
#2330=ORIENTED_EDGE('',*,*,#1762,.F.);
#2331=ORIENTED_EDGE('',*,*,#1749,.F.);
#2332=ORIENTED_EDGE('',*,*,#1762,.T.);
#2333=ORIENTED_EDGE('',*,*,#1728,.F.);
#2334=ORIENTED_EDGE('',*,*,#1759,.F.);
#2335=ORIENTED_EDGE('',*,*,#1750,.F.);
#3002=PLANE('',#3380);
#3003=PLANE('',#3381);
#3004=PLANE('',#3382);
#3005=PLANE('',#3383);
#3006=PLANE('',#3384);
#3007=PLANE('',#3389);
#3008=PLANE('',#3390);
#3009=PLANE('',#3391);
#3010=PLANE('',#3396);
#3011=PLANE('',#3397);
#3012=PLANE('',#3398);
#3013=PLANE('',#3403);
#3014=PLANE('',#3408);
#3015=PLANE('',#3411);
#3016=PLANE('',#3416);
#3017=PLANE('',#3419);
#3018=PLANE('',#3420);
#3019=PLANE('',#3421);
#3020=PLANE('',#3422);
#3021=PLANE('',#3423);
#3022=PLANE('',#3424);
#3023=PLANE('',#3425);
#3024=PLANE('',#3426);
#3025=PLANE('',#3427);
#3026=PLANE('',#3428);
#3027=PLANE('',#3429);
#3028=PLANE('',#3430);
#3029=PLANE('',#3431);
#3030=PLANE('',#3432);
#3031=PLANE('',#3433);
#3032=PLANE('',#3434);
#3033=PLANE('',#3435);
#3127=ADVANCED_FACE('',(#236),#3002,.T.);
#3128=ADVANCED_FACE('',(#237),#3003,.T.);
#3129=ADVANCED_FACE('',(#238),#3004,.F.);
#3130=ADVANCED_FACE('',(#239),#3005,.F.);
#3131=ADVANCED_FACE('',(#240),#3006,.T.);
#3132=ADVANCED_FACE('',(#241),#3007,.T.);
#3133=ADVANCED_FACE('',(#242),#3008,.T.);
#3134=ADVANCED_FACE('',(#243),#3009,.T.);
#3135=ADVANCED_FACE('',(#244),#3010,.T.);
#3136=ADVANCED_FACE('',(#245),#3011,.T.);
#3137=ADVANCED_FACE('',(#246),#3012,.T.);
#3138=ADVANCED_FACE('',(#247),#113,.T.);
#3139=ADVANCED_FACE('',(#248),#114,.T.);
#3140=ADVANCED_FACE('',(#249,#80,#81),#3013,.T.);
#3141=ADVANCED_FACE('',(#250),#115,.T.);
#3142=ADVANCED_FACE('',(#251),#116,.T.);
#3143=ADVANCED_FACE('',(#252),#3014,.T.);
#3144=ADVANCED_FACE('',(#253),#3015,.T.);
#3145=ADVANCED_FACE('',(#254),#117,.F.);
#3146=ADVANCED_FACE('',(#255),#118,.F.);
#3147=ADVANCED_FACE('',(#256),#3016,.T.);
#3148=ADVANCED_FACE('',(#257),#119,.F.);
#3149=ADVANCED_FACE('',(#258),#120,.F.);
#3150=ADVANCED_FACE('',(#259,#82,#83),#3017,.T.);
#3151=ADVANCED_FACE('',(#260),#3018,.F.);
#3152=ADVANCED_FACE('',(#261),#3019,.T.);
#3153=ADVANCED_FACE('',(#262),#3020,.T.);
#3154=ADVANCED_FACE('',(#263),#3021,.T.);
#3155=ADVANCED_FACE('',(#264),#3022,.T.);
#3156=ADVANCED_FACE('',(#265),#3023,.F.);
#3157=ADVANCED_FACE('',(#266),#3024,.F.);
#3158=ADVANCED_FACE('',(#267),#3025,.T.);
#3159=ADVANCED_FACE('',(#268),#3026,.F.);
#3160=ADVANCED_FACE('',(#269),#3027,.F.);
#3161=ADVANCED_FACE('',(#270),#3028,.T.);
#3162=ADVANCED_FACE('',(#271),#3029,.F.);
#3163=ADVANCED_FACE('',(#272),#3030,.F.);
#3164=ADVANCED_FACE('',(#273),#3031,.F.);
#3165=ADVANCED_FACE('',(#274),#3032,.T.);
#3166=ADVANCED_FACE('',(#275),#3033,.T.);
#3293=CLOSED_SHELL('',(#3127,#3128,#3129,#3130,#3131,#3132,#3133,#3134,
#3135,#3136,#3137,#3138,#3139,#3140,#3141,#3142,#3143,#3144,#3145,#3146,
#3147,#3148,#3149,#3150,#3151,#3152,#3153,#3154,#3155,#3156,#3157,#3158,
#3159,#3160,#3161,#3162,#3163,#3164,#3165,#3166));
#3379=AXIS2_PLACEMENT_3D('',#4550,#3647,#3648);
#3380=AXIS2_PLACEMENT_3D('',#4551,#3649,#3650);
#3381=AXIS2_PLACEMENT_3D('',#4560,#3655,#3656);
#3382=AXIS2_PLACEMENT_3D('',#4566,#3660,#3661);
#3383=AXIS2_PLACEMENT_3D('',#4572,#3665,#3666);
#3384=AXIS2_PLACEMENT_3D('',#4575,#3669,#3670);
#3385=AXIS2_PLACEMENT_3D('',#4584,#3674,#3675);
#3386=AXIS2_PLACEMENT_3D('',#4588,#3677,#3678);
#3387=AXIS2_PLACEMENT_3D('',#4596,#3682,#3683);
#3388=AXIS2_PLACEMENT_3D('',#4599,#3685,#3686);
#3389=AXIS2_PLACEMENT_3D('',#4600,#3687,#3688);
#3390=AXIS2_PLACEMENT_3D('',#4622,#3700,#3701);
#3391=AXIS2_PLACEMENT_3D('',#4644,#3713,#3714);
#3392=AXIS2_PLACEMENT_3D('',#4650,#3717,#3718);
#3393=AXIS2_PLACEMENT_3D('',#4654,#3720,#3721);
#3394=AXIS2_PLACEMENT_3D('',#4659,#3724,#3725);
#3395=AXIS2_PLACEMENT_3D('',#4662,#3727,#3728);
#3396=AXIS2_PLACEMENT_3D('',#4663,#3729,#3730);
#3397=AXIS2_PLACEMENT_3D('',#4682,#3741,#3742);
#3398=AXIS2_PLACEMENT_3D('',#4701,#3753,#3754);
#3399=AXIS2_PLACEMENT_3D('',#4707,#3758,#3759);
#3400=AXIS2_PLACEMENT_3D('',#4708,#3760,#3761);
#3401=AXIS2_PLACEMENT_3D('',#4709,#3762,#3763);
#3402=AXIS2_PLACEMENT_3D('',#4712,#3765,#3766);
#3403=AXIS2_PLACEMENT_3D('',#4713,#3767,#3768);
#3404=AXIS2_PLACEMENT_3D('',#4725,#3775,#3776);
#3405=AXIS2_PLACEMENT_3D('',#4726,#3777,#3778);
#3406=AXIS2_PLACEMENT_3D('',#4727,#3779,#3780);
#3407=AXIS2_PLACEMENT_3D('',#4728,#3781,#3782);
#3408=AXIS2_PLACEMENT_3D('',#4729,#3783,#3784);
#3409=AXIS2_PLACEMENT_3D('',#4733,#3787,#3788);
#3410=AXIS2_PLACEMENT_3D('',#4736,#3790,#3791);
#3411=AXIS2_PLACEMENT_3D('',#4737,#3792,#3793);
#3412=AXIS2_PLACEMENT_3D('',#4740,#3795,#3796);
#3413=AXIS2_PLACEMENT_3D('',#4743,#3798,#3799);
#3414=AXIS2_PLACEMENT_3D('',#4745,#3801,#3802);
#3415=AXIS2_PLACEMENT_3D('',#4747,#3804,#3805);
#3416=AXIS2_PLACEMENT_3D('',#4749,#3807,#3808);
#3417=AXIS2_PLACEMENT_3D('',#4751,#3810,#3811);
#3418=AXIS2_PLACEMENT_3D('',#4752,#3812,#3813);
#3419=AXIS2_PLACEMENT_3D('',#4754,#3815,#3816);
#3420=AXIS2_PLACEMENT_3D('',#4763,#3821,#3822);
#3421=AXIS2_PLACEMENT_3D('',#4765,#3824,#3825);
#3422=AXIS2_PLACEMENT_3D('',#4767,#3827,#3828);
#3423=AXIS2_PLACEMENT_3D('',#4768,#3829,#3830);
#3424=AXIS2_PLACEMENT_3D('',#4770,#3832,#3833);
#3425=AXIS2_PLACEMENT_3D('',#4772,#3835,#3836);
#3426=AXIS2_PLACEMENT_3D('',#4773,#3837,#3838);
#3427=AXIS2_PLACEMENT_3D('',#4775,#3840,#3841);
#3428=AXIS2_PLACEMENT_3D('',#4777,#3843,#3844);
#3429=AXIS2_PLACEMENT_3D('',#4778,#3845,#3846);
#3430=AXIS2_PLACEMENT_3D('',#4780,#3848,#3849);
#3431=AXIS2_PLACEMENT_3D('',#4782,#3851,#3852);
#3432=AXIS2_PLACEMENT_3D('',#4783,#3853,#3854);
#3433=AXIS2_PLACEMENT_3D('',#4786,#3857,#3858);
#3434=AXIS2_PLACEMENT_3D('',#4788,#3860,#3861);
#3435=AXIS2_PLACEMENT_3D('',#4790,#3863,#3864);
#3647=DIRECTION('axis',(0.,0.,1.));
#3648=DIRECTION('refdir',(1.,0.,0.));
#3649=DIRECTION('center_axis',(0.,-1.,-5.78241158658936E-16));
#3650=DIRECTION('ref_axis',(0.,5.78241158658936E-16,-1.));
#3651=DIRECTION('',(-3.06161699786839E-16,-5.78241158658936E-16,1.));
#3652=DIRECTION('',(1.,-1.77035296021731E-31,3.06161699786839E-16));
#3653=DIRECTION('',(-3.06161699786839E-16,-5.78241158658936E-16,1.));
#3654=DIRECTION('',(-1.,1.77035296021731E-31,-3.06161699786839E-16));
#3655=DIRECTION('center_axis',(-1.,-2.73691106313441E-47,-3.06161699786839E-16));
#3656=DIRECTION('ref_axis',(3.06161699786839E-16,0.,-1.));
#3657=DIRECTION('',(1.4960729241273E-31,-1.,-4.88654500275157E-16));
#3658=DIRECTION('',(-3.06161699786839E-16,-5.78241158658936E-16,1.));
#3659=DIRECTION('',(-1.77035296021731E-31,1.,5.78241158658936E-16));
#3660=DIRECTION('center_axis',(0.,-1.,-5.78241158658936E-16));
#3661=DIRECTION('ref_axis',(0.,5.78241158658936E-16,-1.));
#3662=DIRECTION('',(1.,-1.77035296021731E-31,3.06161699786839E-16));
#3663=DIRECTION('',(-3.06161699786839E-16,-5.78241158658936E-16,1.));
#3664=DIRECTION('',(-1.,1.77035296021731E-31,-3.06161699786839E-16));
#3665=DIRECTION('center_axis',(-1.,-2.73691106313441E-47,-3.06161699786839E-16));
#3666=DIRECTION('ref_axis',(3.06161699786839E-16,0.,-1.));
#3667=DIRECTION('',(1.4960729241273E-31,-1.,-4.88654500275157E-16));
#3668=DIRECTION('',(-1.77035296021731E-31,1.,5.78241158658936E-16));
#3669=DIRECTION('center_axis',(1.,0.,0.));
#3670=DIRECTION('ref_axis',(0.,1.,0.));
#3671=DIRECTION('',(0.,5.78241158658936E-16,-1.));
#3672=DIRECTION('',(0.,1.,0.));
#3673=DIRECTION('',(0.,0.,1.));
#3674=DIRECTION('center_axis',(1.,0.,0.));
#3675=DIRECTION('ref_axis',(0.,0.,-1.));
#3676=DIRECTION('',(0.,1.,4.88654500275157E-16));
#3677=DIRECTION('center_axis',(1.,0.,0.));
#3678=DIRECTION('ref_axis',(0.,0.,-1.));
#3679=DIRECTION('',(0.,-4.88654500275157E-16,1.));
#3680=DIRECTION('',(0.,1.,0.));
#3681=DIRECTION('',(0.,-5.78241158658936E-16,1.));
#3682=DIRECTION('center_axis',(1.,0.,0.));
#3683=DIRECTION('ref_axis',(0.,0.,-1.));
#3684=DIRECTION('',(0.,-1.,-5.78241158658936E-16));
#3685=DIRECTION('center_axis',(1.,0.,0.));
#3686=DIRECTION('ref_axis',(0.,0.,-1.));
#3687=DIRECTION('center_axis',(-1.4960729241273E-31,-1.,-4.88654500275157E-16));
#3688=DIRECTION('ref_axis',(9.30044539122197E-64,4.88654500275157E-16,-1.));
#3689=DIRECTION('',(1.,-1.4960729241273E-31,0.));
#3690=DIRECTION('',(-2.8256014442301E-31,4.88654500275157E-16,-1.));
#3691=DIRECTION('',(1.,-1.4960729241273E-31,0.));
#3692=DIRECTION('',(1.,0.,-3.06161699786839E-16));
#3693=DIRECTION('',(-1.22464679914735E-16,4.88654500275157E-16,-1.));
#3694=DIRECTION('',(-1.,1.4960729241273E-31,0.));
#3695=DIRECTION('',(2.8256014442301E-31,4.88654500275157E-16,-1.));
#3696=DIRECTION('',(-1.,1.4960729241273E-31,0.));
#3697=DIRECTION('',(-1.22464679914735E-16,4.88654500275157E-16,-1.));
#3698=DIRECTION('',(1.,0.,-3.06161699786839E-16));
#3699=DIRECTION('',(0.,-4.88654500275157E-16,1.));
#3700=DIRECTION('center_axis',(0.,1.,0.));
#3701=DIRECTION('ref_axis',(0.,0.,1.));
#3702=DIRECTION('',(-1.,0.,0.));
#3703=DIRECTION('',(0.,0.,1.));
#3704=DIRECTION('',(1.,0.,-3.06161699786839E-16));
#3705=DIRECTION('',(-1.22464679914735E-16,0.,-1.));
#3706=DIRECTION('',(1.,0.,0.));
#3707=DIRECTION('',(0.,0.,1.));
#3708=DIRECTION('',(1.,0.,0.));
#3709=DIRECTION('',(-1.22464679914735E-16,0.,-1.));
#3710=DIRECTION('',(1.,0.,-3.06161699786839E-16));
#3711=DIRECTION('',(-1.,0.,0.));
#3712=DIRECTION('',(0.,0.,1.));
#3713=DIRECTION('center_axis',(-1.,0.,1.22464679914735E-16));
#3714=DIRECTION('ref_axis',(0.,-1.,0.));
#3715=DIRECTION('',(0.,1.,0.));
#3716=DIRECTION('',(-1.22464679914735E-16,5.78241158658936E-16,-1.));
#3717=DIRECTION('center_axis',(-1.,0.,1.22464679914735E-16));
#3718=DIRECTION('ref_axis',(1.22464679914735E-16,0.,1.));
#3719=DIRECTION('',(-7.08141184086923E-32,-1.,-5.78241158658936E-16));
#3720=DIRECTION('center_axis',(-1.,0.,1.22464679914735E-16));
#3721=DIRECTION('ref_axis',(1.22464679914735E-16,0.,1.));
#3722=DIRECTION('',(1.22464679914735E-16,-5.78241158658936E-16,1.));
#3723=DIRECTION('',(0.,1.,0.));
#3724=DIRECTION('center_axis',(-1.,0.,1.22464679914735E-16));
#3725=DIRECTION('ref_axis',(1.22464679914735E-16,0.,1.));
#3726=DIRECTION('',(-5.9842916965092E-32,-1.,-4.88654500275157E-16));
#3727=DIRECTION('center_axis',(-1.,0.,1.22464679914735E-16));
#3728=DIRECTION('ref_axis',(1.22464679914735E-16,0.,1.));
#3729=DIRECTION('center_axis',(1.77035296021731E-31,1.,5.78241158658936E-16));
#3730=DIRECTION('ref_axis',(6.82567686290692E-63,-5.78241158658936E-16,
1.));
#3731=DIRECTION('',(-1.,1.77035296021731E-31,0.));
#3732=DIRECTION('',(0.,-5.78241158658936E-16,1.));
#3733=DIRECTION('',(1.,0.,-3.06161699786839E-16));
#3734=DIRECTION('',(1.,-1.77035296021731E-31,0.));
#3735=DIRECTION('',(-3.34362837567229E-31,-5.78241158658936E-16,1.));
#3736=DIRECTION('',(1.,-1.77035296021731E-31,0.));
#3737=DIRECTION('',(-1.22464679914735E-16,5.78241158658936E-16,-1.));
#3738=DIRECTION('',(1.,0.,-3.06161699786839E-16));
#3739=DIRECTION('',(-1.,1.77035296021731E-31,0.));
#3740=DIRECTION('',(3.34362837567229E-31,-5.78241158658936E-16,1.));
#3741=DIRECTION('center_axis',(-1.77035296021731E-31,-1.,-5.78241158658936E-16));
#3742=DIRECTION('ref_axis',(-6.82567686290692E-63,5.78241158658936E-16,
-1.));
#3743=DIRECTION('',(1.,-1.77035296021731E-31,0.));
#3744=DIRECTION('',(-3.34362837567229E-31,5.78241158658936E-16,-1.));
#3745=DIRECTION('',(1.,-1.77035296021731E-31,0.));
#3746=DIRECTION('',(1.,0.,-3.06161699786839E-16));
#3747=DIRECTION('',(1.22464679914735E-16,-5.78241158658936E-16,1.));
#3748=DIRECTION('',(-1.,1.77035296021731E-31,0.));
#3749=DIRECTION('',(3.34362837567229E-31,5.78241158658936E-16,-1.));
#3750=DIRECTION('',(-1.,1.77035296021731E-31,0.));
#3751=DIRECTION('',(1.,0.,-3.06161699786839E-16));
#3752=DIRECTION('',(0.,5.78241158658936E-16,-1.));
#3753=DIRECTION('center_axis',(-3.06161699786839E-16,5.78241158658936E-16,
-1.));
#3754=DIRECTION('ref_axis',(0.,1.,5.78241158658936E-16));
#3755=DIRECTION('',(0.,1.,5.78241158658936E-16));
#3756=DIRECTION('',(1.,0.,-3.06161699786839E-16));
#3757=DIRECTION('',(1.,0.,-3.06161699786839E-16));
#3758=DIRECTION('center_axis',(1.,0.,-3.06161699786839E-16));
#3759=DIRECTION('ref_axis',(-3.06161699786839E-16,0.,-1.));
#3760=DIRECTION('center_axis',(1.,0.,0.));
#3761=DIRECTION('ref_axis',(0.,0.,-1.));
#3762=DIRECTION('center_axis',(1.,0.,-3.06161699786839E-16));
#3763=DIRECTION('ref_axis',(-3.06161699786839E-16,0.,-1.));
#3764=DIRECTION('',(1.,0.,-3.06161699786839E-16));
#3765=DIRECTION('center_axis',(-1.,0.,1.22464679914735E-16));
#3766=DIRECTION('ref_axis',(1.22464679914735E-16,0.,1.));
#3767=DIRECTION('center_axis',(3.06161699786839E-16,-5.78241158658936E-16,
1.));
#3768=DIRECTION('ref_axis',(0.,-1.,-5.78241158658936E-16));
#3769=DIRECTION('',(1.,0.,-3.06161699786839E-16));
#3770=DIRECTION('',(7.08141184086923E-32,1.,5.78241158658936E-16));
#3771=DIRECTION('',(1.,1.77035296021731E-31,-3.06161699786839E-16));
#3772=DIRECTION('',(1.77035296021731E-31,1.,5.78241158658936E-16));
#3773=DIRECTION('',(1.,1.77035296021731E-31,-3.06161699786839E-16));
#3774=DIRECTION('',(1.77035296021731E-31,1.,5.78241158658936E-16));
#3775=DIRECTION('center_axis',(1.,0.,-3.06161699786839E-16));
#3776=DIRECTION('ref_axis',(-3.06161699786839E-16,0.,-1.));
#3777=DIRECTION('center_axis',(-1.,0.,1.22464679914735E-16));
#3778=DIRECTION('ref_axis',(1.22464679914735E-16,0.,1.));
#3779=DIRECTION('center_axis',(1.,0.,-3.06161699786839E-16));
#3780=DIRECTION('ref_axis',(-3.06161699786839E-16,0.,-1.));
#3781=DIRECTION('center_axis',(1.,0.,0.));
#3782=DIRECTION('ref_axis',(0.,0.,-1.));
#3783=DIRECTION('center_axis',(1.,0.,0.));
#3784=DIRECTION('ref_axis',(0.,1.,0.));
#3785=DIRECTION('',(0.,1.,0.));
#3786=DIRECTION('',(0.,1.,0.));
#3787=DIRECTION('center_axis',(1.,0.,0.));
#3788=DIRECTION('ref_axis',(0.,0.,-1.));
#3789=DIRECTION('',(0.,1.,4.88654500275157E-16));
#3790=DIRECTION('center_axis',(1.,0.,0.));
#3791=DIRECTION('ref_axis',(0.,0.,-1.));
#3792=DIRECTION('center_axis',(-1.,0.,1.22464679914735E-16));
#3793=DIRECTION('ref_axis',(0.,-1.,0.));
#3794=DIRECTION('',(0.,1.,0.));
#3795=DIRECTION('center_axis',(-1.,0.,1.22464679914735E-16));
#3796=DIRECTION('ref_axis',(1.22464679914735E-16,0.,1.));
#3797=DIRECTION('',(-5.98429169650921E-32,-1.,-4.88654500275157E-16));
#3798=DIRECTION('center_axis',(-1.,0.,1.22464679914735E-16));
#3799=DIRECTION('ref_axis',(1.22464679914735E-16,0.,1.));
#3800=DIRECTION('',(0.,1.,0.));
#3801=DIRECTION('center_axis',(1.,0.,-3.06161699786839E-16));
#3802=DIRECTION('ref_axis',(-3.06161699786839E-16,0.,-1.));
#3803=DIRECTION('',(1.,0.,-3.06161699786839E-16));
#3804=DIRECTION('center_axis',(1.,0.,-3.06161699786839E-16));
#3805=DIRECTION('ref_axis',(-3.06161699786839E-16,0.,-1.));
#3806=DIRECTION('',(1.,0.,-3.06161699786839E-16));
#3807=DIRECTION('center_axis',(3.06161699786839E-16,-4.88654500275157E-16,
1.));
#3808=DIRECTION('ref_axis',(0.,-1.,-4.88654500275157E-16));
#3809=DIRECTION('',(1.,0.,-3.06161699786839E-16));
#3810=DIRECTION('center_axis',(1.,0.,-3.06161699786839E-16));
#3811=DIRECTION('ref_axis',(-3.06161699786839E-16,0.,-1.));
#3812=DIRECTION('center_axis',(1.,0.,-3.06161699786839E-16));
#3813=DIRECTION('ref_axis',(-3.06161699786839E-16,0.,-1.));
#3814=DIRECTION('',(1.,0.,-3.06161699786839E-16));
#3815=DIRECTION('center_axis',(-3.06161699786839E-16,4.88654500275157E-16,
-1.));
#3816=DIRECTION('ref_axis',(0.,1.,4.88654500275157E-16));
#3817=DIRECTION('',(-1.,-1.77035296021731E-31,3.06161699786839E-16));
#3818=DIRECTION('',(-1.4960729241273E-31,-1.,-4.88654500275157E-16));
#3819=DIRECTION('',(-1.,-1.77035296021731E-31,3.06161699786839E-16));
#3820=DIRECTION('',(-1.4960729241273E-31,-1.,-4.88654500275157E-16));
#3821=DIRECTION('center_axis',(0.,0.,1.));
#3822=DIRECTION('ref_axis',(1.,0.,0.));
#3823=DIRECTION('',(-5.78241158658936E-16,-1.,0.));
#3824=DIRECTION('center_axis',(-1.,5.78241158658936E-16,0.));
#3825=DIRECTION('ref_axis',(-5.78241158658936E-16,-1.,0.));
#3826=DIRECTION('',(-5.78241158658936E-16,-1.,0.));
#3827=DIRECTION('center_axis',(0.,0.,1.));
#3828=DIRECTION('ref_axis',(1.,0.,0.));
#3829=DIRECTION('center_axis',(0.,0.,1.));
#3830=DIRECTION('ref_axis',(1.,0.,0.));
#3831=DIRECTION('',(-5.78241158658936E-16,-1.,0.));
#3832=DIRECTION('center_axis',(-1.,5.78241158658936E-16,0.));
#3833=DIRECTION('ref_axis',(-5.78241158658936E-16,-1.,0.));
#3834=DIRECTION('',(-5.78241158658936E-16,-1.,0.));
#3835=DIRECTION('center_axis',(0.,0.,1.));
#3836=DIRECTION('ref_axis',(1.,0.,0.));
#3837=DIRECTION('center_axis',(0.,0.,-1.));
#3838=DIRECTION('ref_axis',(-1.,0.,0.));
#3839=DIRECTION('',(5.78241158658936E-16,-1.,0.));
#3840=DIRECTION('center_axis',(0.,0.,-1.));
#3841=DIRECTION('ref_axis',(-1.,0.,0.));
#3842=DIRECTION('',(5.78241158658936E-16,-1.,0.));
#3843=DIRECTION('center_axis',(-1.,-5.78241158658936E-16,0.));
#3844=DIRECTION('ref_axis',(5.78241158658936E-16,-1.,0.));
#3845=DIRECTION('center_axis',(0.,0.,-1.));
#3846=DIRECTION('ref_axis',(-1.,0.,0.));
#3847=DIRECTION('',(5.78241158658936E-16,-1.,0.));
#3848=DIRECTION('center_axis',(0.,0.,-1.));
#3849=DIRECTION('ref_axis',(-1.,0.,0.));
#3850=DIRECTION('',(5.78241158658936E-16,-1.,0.));
#3851=DIRECTION('center_axis',(-1.,-5.78241158658936E-16,0.));
#3852=DIRECTION('ref_axis',(5.78241158658936E-16,-1.,0.));
#3853=DIRECTION('center_axis',(0.,-1.,-5.78241158658936E-16));
#3854=DIRECTION('ref_axis',(0.,5.78241158658936E-16,-1.));
#3855=DIRECTION('',(3.06161699786839E-16,-5.78241158658936E-16,1.));
#3856=DIRECTION('',(3.06161699786839E-16,-5.78241158658936E-16,1.));
#3857=DIRECTION('center_axis',(1.,-2.73691106313441E-47,-3.06161699786839E-16));
#3858=DIRECTION('ref_axis',(-3.06161699786839E-16,0.,-1.));
#3859=DIRECTION('',(3.06161699786839E-16,-5.78241158658936E-16,1.));
#3860=DIRECTION('center_axis',(0.,-1.,-5.78241158658936E-16));
#3861=DIRECTION('ref_axis',(0.,5.78241158658936E-16,-1.));
#3862=DIRECTION('',(3.06161699786839E-16,-5.78241158658936E-16,1.));
#3863=DIRECTION('center_axis',(1.,-2.73691106313441E-47,-3.06161699786839E-16));
#3864=DIRECTION('ref_axis',(-3.06161699786839E-16,0.,-1.));
#4550=CARTESIAN_POINT('',(0.,0.,0.));
#4551=CARTESIAN_POINT('Origin',(155.,858.5,147.));
#4552=CARTESIAN_POINT('',(151.,858.5,168.));
#4553=CARTESIAN_POINT('',(151.,858.5,172.));
#4554=CARTESIAN_POINT('',(151.,858.5,147.));
#4555=CARTESIAN_POINT('',(159.,858.5,168.));
#4556=CARTESIAN_POINT('',(360.,858.5,168.));
#4557=CARTESIAN_POINT('',(159.,858.5,172.));
#4558=CARTESIAN_POINT('',(159.,858.5,147.));
#4559=CARTESIAN_POINT('',(155.,858.5,172.));
#4560=CARTESIAN_POINT('Origin',(159.,850.,147.));
#4561=CARTESIAN_POINT('',(159.,841.5,168.));
#4562=CARTESIAN_POINT('',(159.,850.,168.));
#4563=CARTESIAN_POINT('',(159.,841.5,172.));
#4564=CARTESIAN_POINT('',(159.,841.5,147.));
#4565=CARTESIAN_POINT('',(159.,850.,172.));
#4566=CARTESIAN_POINT('Origin',(155.,841.5,147.));
#4567=CARTESIAN_POINT('',(151.,841.5,168.));
#4568=CARTESIAN_POINT('',(360.,841.5,168.));
#4569=CARTESIAN_POINT('',(151.,841.5,172.));
#4570=CARTESIAN_POINT('',(151.,841.5,147.));
#4571=CARTESIAN_POINT('',(155.,841.5,172.));
#4572=CARTESIAN_POINT('Origin',(151.,850.,147.));
#4573=CARTESIAN_POINT('',(151.,850.,168.));
#4574=CARTESIAN_POINT('',(151.,850.,172.));
#4575=CARTESIAN_POINT('Origin',(380.,850.,152.));
#4576=CARTESIAN_POINT('',(380.,830.,170.));
#4577=CARTESIAN_POINT('',(380.,830.,158.));
#4578=CARTESIAN_POINT('',(380.,830.,152.));
#4579=CARTESIAN_POINT('',(380.,834.,158.));
#4580=CARTESIAN_POINT('',(380.,850.,158.));
#4581=CARTESIAN_POINT('',(380.,834.,166.2));
#4582=CARTESIAN_POINT('',(380.,834.,152.));
#4583=CARTESIAN_POINT('',(380.,835.8,168.));
#4584=CARTESIAN_POINT('Origin',(380.,835.8,166.2));
#4585=CARTESIAN_POINT('',(380.,864.2,168.));
#4586=CARTESIAN_POINT('',(380.,850.,168.));
#4587=CARTESIAN_POINT('',(380.,866.,166.2));
#4588=CARTESIAN_POINT('Origin',(380.,864.2,166.2));
#4589=CARTESIAN_POINT('',(380.,866.,158.));
#4590=CARTESIAN_POINT('',(380.,866.,152.));
#4591=CARTESIAN_POINT('',(380.,870.,158.));
#4592=CARTESIAN_POINT('',(380.,850.,158.));
#4593=CARTESIAN_POINT('',(380.,870.,170.));
#4594=CARTESIAN_POINT('',(380.,870.,152.));
#4595=CARTESIAN_POINT('',(380.,868.,172.));
#4596=CARTESIAN_POINT('Origin',(380.,868.,170.));
#4597=CARTESIAN_POINT('',(380.,832.,172.));
#4598=CARTESIAN_POINT('',(380.,850.,172.));
#4599=CARTESIAN_POINT('Origin',(380.,832.,170.));
#4600=CARTESIAN_POINT('Origin',(-360.,866.,152.));
#4601=CARTESIAN_POINT('',(375.,866.,146.));
#4602=CARTESIAN_POINT('',(380.,866.,146.));
#4603=CARTESIAN_POINT('',(-360.,866.,146.));
#4604=CARTESIAN_POINT('',(375.,866.,158.));
#4605=CARTESIAN_POINT('',(375.,866.,152.));
#4606=CARTESIAN_POINT('',(-360.,866.,158.));
#4607=CARTESIAN_POINT('',(-380.,866.,166.2));
#4608=CARTESIAN_POINT('',(-360.,866.,166.2));
#4609=CARTESIAN_POINT('',(-380.,866.,158.));
#4610=CARTESIAN_POINT('',(-380.,866.,152.));
#4611=CARTESIAN_POINT('',(-375.,866.,158.));
#4612=CARTESIAN_POINT('',(-360.,866.,158.));
#4613=CARTESIAN_POINT('',(-375.,866.,146.));
#4614=CARTESIAN_POINT('',(-375.,866.,152.));
#4615=CARTESIAN_POINT('',(-380.,866.,146.));
#4616=CARTESIAN_POINT('',(-360.,866.,146.));
#4617=CARTESIAN_POINT('',(-380.,866.,137.8));
#4618=CARTESIAN_POINT('',(-380.,866.,152.));
#4619=CARTESIAN_POINT('',(380.,866.,137.8));
#4620=CARTESIAN_POINT('',(-360.,866.,137.8));
#4621=CARTESIAN_POINT('',(380.,866.,152.));
#4622=CARTESIAN_POINT('Origin',(-360.,834.,152.));
#4623=CARTESIAN_POINT('',(380.,834.,146.));
#4624=CARTESIAN_POINT('',(375.,834.,146.));
#4625=CARTESIAN_POINT('',(-360.,834.,146.));
#4626=CARTESIAN_POINT('',(380.,834.,137.8));
#4627=CARTESIAN_POINT('',(380.,834.,152.));
#4628=CARTESIAN_POINT('',(-380.,834.,137.8));
#4629=CARTESIAN_POINT('',(-360.,834.,137.8));
#4630=CARTESIAN_POINT('',(-380.,834.,146.));
#4631=CARTESIAN_POINT('',(-380.,834.,152.));
#4632=CARTESIAN_POINT('',(-375.,834.,146.));
#4633=CARTESIAN_POINT('',(-360.,834.,146.));
#4634=CARTESIAN_POINT('',(-375.,834.,158.));
#4635=CARTESIAN_POINT('',(-375.,834.,152.));
#4636=CARTESIAN_POINT('',(-380.,834.,158.));
#4637=CARTESIAN_POINT('',(-360.,834.,158.));
#4638=CARTESIAN_POINT('',(-380.,834.,166.2));
#4639=CARTESIAN_POINT('',(-380.,834.,152.));
#4640=CARTESIAN_POINT('',(-360.,834.,166.2));
#4641=CARTESIAN_POINT('',(375.,834.,158.));
#4642=CARTESIAN_POINT('',(-360.,834.,158.));
#4643=CARTESIAN_POINT('',(375.,834.,152.));
#4644=CARTESIAN_POINT('Origin',(-380.,850.,152.));
#4645=CARTESIAN_POINT('',(-380.,870.,146.));
#4646=CARTESIAN_POINT('',(-380.,850.,146.));
#4647=CARTESIAN_POINT('',(-380.,870.,134.));
#4648=CARTESIAN_POINT('',(-380.,870.,152.));
#4649=CARTESIAN_POINT('',(-380.,868.,132.));
#4650=CARTESIAN_POINT('Origin',(-380.,868.,134.));
#4651=CARTESIAN_POINT('',(-380.,832.,132.));
#4652=CARTESIAN_POINT('',(-380.,850.,132.));
#4653=CARTESIAN_POINT('',(-380.,830.,134.));
#4654=CARTESIAN_POINT('Origin',(-380.,832.,134.));
#4655=CARTESIAN_POINT('',(-380.,830.,146.));
#4656=CARTESIAN_POINT('',(-380.,830.,152.));
#4657=CARTESIAN_POINT('',(-380.,850.,146.));
#4658=CARTESIAN_POINT('',(-380.,835.8,136.));
#4659=CARTESIAN_POINT('Origin',(-380.,835.8,137.8));
#4660=CARTESIAN_POINT('',(-380.,864.2,136.));
#4661=CARTESIAN_POINT('',(-380.,850.,136.));
#4662=CARTESIAN_POINT('Origin',(-380.,864.2,137.8));
#4663=CARTESIAN_POINT('Origin',(-360.,870.,152.));
#4664=CARTESIAN_POINT('',(380.,870.,146.));
#4665=CARTESIAN_POINT('',(375.,870.,146.));
#4666=CARTESIAN_POINT('',(-360.,870.,146.));
#4667=CARTESIAN_POINT('',(380.,870.,134.));
#4668=CARTESIAN_POINT('',(380.,870.,152.));
#4669=CARTESIAN_POINT('',(-360.,870.,134.));
#4670=CARTESIAN_POINT('',(-375.,870.,146.));
#4671=CARTESIAN_POINT('',(-360.,870.,146.));
#4672=CARTESIAN_POINT('',(-375.,870.,158.));
#4673=CARTESIAN_POINT('',(-375.,870.,152.));
#4674=CARTESIAN_POINT('',(-380.,870.,158.));
#4675=CARTESIAN_POINT('',(-360.,870.,158.));
#4676=CARTESIAN_POINT('',(-380.,870.,170.));
#4677=CARTESIAN_POINT('',(-380.,870.,152.));
#4678=CARTESIAN_POINT('',(-360.,870.,170.));
#4679=CARTESIAN_POINT('',(375.,870.,158.));
#4680=CARTESIAN_POINT('',(-360.,870.,158.));
#4681=CARTESIAN_POINT('',(375.,870.,152.));
#4682=CARTESIAN_POINT('Origin',(-360.,830.,152.));
#4683=CARTESIAN_POINT('',(375.,830.,146.));
#4684=CARTESIAN_POINT('',(380.,830.,146.));
#4685=CARTESIAN_POINT('',(-360.,830.,146.));
#4686=CARTESIAN_POINT('',(375.,830.,158.));
#4687=CARTESIAN_POINT('',(375.,830.,152.));
#4688=CARTESIAN_POINT('',(-360.,830.,158.));
#4689=CARTESIAN_POINT('',(-380.,830.,170.));
#4690=CARTESIAN_POINT('',(-360.,830.,170.));
#4691=CARTESIAN_POINT('',(-380.,830.,158.));
#4692=CARTESIAN_POINT('',(-380.,830.,152.));
#4693=CARTESIAN_POINT('',(-375.,830.,158.));
#4694=CARTESIAN_POINT('',(-360.,830.,158.));
#4695=CARTESIAN_POINT('',(-375.,830.,146.));
#4696=CARTESIAN_POINT('',(-375.,830.,152.));
#4697=CARTESIAN_POINT('',(-360.,830.,146.));
#4698=CARTESIAN_POINT('',(380.,830.,134.));
#4699=CARTESIAN_POINT('',(-360.,830.,134.));
#4700=CARTESIAN_POINT('',(380.,830.,152.));
#4701=CARTESIAN_POINT('Origin',(-360.,850.,132.));
#4702=CARTESIAN_POINT('',(380.,832.,132.));
#4703=CARTESIAN_POINT('',(380.,868.,132.));
#4704=CARTESIAN_POINT('',(380.,850.,132.));
#4705=CARTESIAN_POINT('',(-360.,832.,132.));
#4706=CARTESIAN_POINT('',(-360.,868.,132.));
#4707=CARTESIAN_POINT('Origin',(-360.,832.,134.));
#4708=CARTESIAN_POINT('Origin',(380.,832.,134.));
#4709=CARTESIAN_POINT('Origin',(-360.,832.,170.));
#4710=CARTESIAN_POINT('',(-380.,832.,172.));
#4711=CARTESIAN_POINT('',(-360.,832.,172.));
#4712=CARTESIAN_POINT('Origin',(-380.,832.,170.));
#4713=CARTESIAN_POINT('Origin',(-360.,850.,172.));
#4714=CARTESIAN_POINT('',(-380.,868.,172.));
#4715=CARTESIAN_POINT('',(-360.,868.,172.));
#4716=CARTESIAN_POINT('',(-380.,850.,172.));
#4717=CARTESIAN_POINT('',(-159.,841.5,172.));
#4718=CARTESIAN_POINT('',(-151.,841.5,172.));
#4719=CARTESIAN_POINT('',(-155.,841.5,172.));
#4720=CARTESIAN_POINT('',(-159.,858.5,172.));
#4721=CARTESIAN_POINT('',(-159.,850.,172.));
#4722=CARTESIAN_POINT('',(-151.,858.5,172.));
#4723=CARTESIAN_POINT('',(-155.,858.5,172.));
#4724=CARTESIAN_POINT('',(-151.,850.,172.));
#4725=CARTESIAN_POINT('Origin',(-360.,868.,170.));
#4726=CARTESIAN_POINT('Origin',(-380.,868.,170.));
#4727=CARTESIAN_POINT('Origin',(-360.,868.,134.));
#4728=CARTESIAN_POINT('Origin',(380.,868.,134.));
#4729=CARTESIAN_POINT('Origin',(380.,850.,152.));
#4730=CARTESIAN_POINT('',(380.,850.,146.));
#4731=CARTESIAN_POINT('',(380.,850.,146.));
#4732=CARTESIAN_POINT('',(380.,864.2,136.));
#4733=CARTESIAN_POINT('Origin',(380.,864.2,137.8));
#4734=CARTESIAN_POINT('',(380.,835.8,136.));
#4735=CARTESIAN_POINT('',(380.,850.,136.));
#4736=CARTESIAN_POINT('Origin',(380.,835.8,137.8));
#4737=CARTESIAN_POINT('Origin',(-380.,850.,152.));
#4738=CARTESIAN_POINT('',(-380.,850.,158.));
#4739=CARTESIAN_POINT('',(-380.,864.2,168.));
#4740=CARTESIAN_POINT('Origin',(-380.,864.2,166.2));
#4741=CARTESIAN_POINT('',(-380.,835.8,168.));
#4742=CARTESIAN_POINT('',(-380.,850.,168.));
#4743=CARTESIAN_POINT('Origin',(-380.,835.8,166.2));
#4744=CARTESIAN_POINT('',(-380.,850.,158.));
#4745=CARTESIAN_POINT('Origin',(-360.,835.8,166.2));
#4746=CARTESIAN_POINT('',(-360.,835.8,168.));
#4747=CARTESIAN_POINT('Origin',(-360.,835.8,137.8));
#4748=CARTESIAN_POINT('',(-360.,835.8,136.));
#4749=CARTESIAN_POINT('Origin',(-360.,850.,136.));
#4750=CARTESIAN_POINT('',(-360.,864.2,136.));
#4751=CARTESIAN_POINT('Origin',(-360.,864.2,137.8));
#4752=CARTESIAN_POINT('Origin',(-360.,864.2,166.2));
#4753=CARTESIAN_POINT('',(-360.,864.2,168.));
#4754=CARTESIAN_POINT('Origin',(-360.,850.,168.));
#4755=CARTESIAN_POINT('',(-151.,841.5,168.));
#4756=CARTESIAN_POINT('',(-159.,841.5,168.));
#4757=CARTESIAN_POINT('',(-360.,841.5,168.));
#4758=CARTESIAN_POINT('',(-151.,858.5,168.));
#4759=CARTESIAN_POINT('',(-151.,850.,168.));
#4760=CARTESIAN_POINT('',(-159.,858.5,168.));
#4761=CARTESIAN_POINT('',(-360.,858.5,168.));
#4762=CARTESIAN_POINT('',(-159.,850.,168.));
#4763=CARTESIAN_POINT('Origin',(-378.,3982.26464896431,158.));
#4764=CARTESIAN_POINT('',(-375.,3982.26464896431,158.));
#4765=CARTESIAN_POINT('Origin',(-375.,3982.26464896431,152.));
#4766=CARTESIAN_POINT('',(-375.,3982.26464896431,146.));
#4767=CARTESIAN_POINT('Origin',(-378.,3982.26464896431,146.));
#4768=CARTESIAN_POINT('Origin',(-378.,3982.26464896431,146.));
#4769=CARTESIAN_POINT('',(-375.,3982.26464896431,146.));
#4770=CARTESIAN_POINT('Origin',(-375.,3982.26464896431,152.));
#4771=CARTESIAN_POINT('',(-375.,3982.26464896431,158.));
#4772=CARTESIAN_POINT('Origin',(-378.,3982.26464896431,158.));
#4773=CARTESIAN_POINT('Origin',(378.,3982.26464896431,146.));
#4774=CARTESIAN_POINT('',(375.,3982.26464896431,146.));
#4775=CARTESIAN_POINT('Origin',(378.,3982.26464896431,158.));
#4776=CARTESIAN_POINT('',(375.,3982.26464896431,158.));
#4777=CARTESIAN_POINT('Origin',(375.,3982.26464896431,152.));
#4778=CARTESIAN_POINT('Origin',(378.,3982.26464896431,146.));
#4779=CARTESIAN_POINT('',(375.,3982.26464896431,146.));
#4780=CARTESIAN_POINT('Origin',(378.,3982.26464896431,158.));
#4781=CARTESIAN_POINT('',(375.,3982.26464896431,158.));
#4782=CARTESIAN_POINT('Origin',(375.,3982.26464896431,152.));
#4783=CARTESIAN_POINT('Origin',(-155.,841.5,147.));
#4784=CARTESIAN_POINT('',(-159.,841.5,147.));
#4785=CARTESIAN_POINT('',(-151.,841.5,147.));
#4786=CARTESIAN_POINT('Origin',(-151.,850.,147.));
#4787=CARTESIAN_POINT('',(-151.,858.5,147.));
#4788=CARTESIAN_POINT('Origin',(-155.,858.5,147.));
#4789=CARTESIAN_POINT('',(-159.,858.5,147.));
#4790=CARTESIAN_POINT('Origin',(-159.,850.,147.));
#5489=UNCERTAINTY_MEASURE_WITH_UNIT(LENGTH_MEASURE(0.01),#5506,
'DISTANCE_ACCURACY_VALUE',
'Maximum model space distance between geometric entities at asserted c
onnectivities');
#5496=UNCERTAINTY_MEASURE_WITH_UNIT(LENGTH_MEASURE(0.01),#5506,
'DISTANCE_ACCURACY_VALUE',
'Maximum model space distance between geometric entities at asserted c
onnectivities');
#5498=(
GEOMETRIC_REPRESENTATION_CONTEXT(3)
GLOBAL_UNCERTAINTY_ASSIGNED_CONTEXT((#5489))
GLOBAL_UNIT_ASSIGNED_CONTEXT((#5506,#5508,#5509))
REPRESENTATION_CONTEXT('','3D')
);
#5505=(
GEOMETRIC_REPRESENTATION_CONTEXT(3)
GLOBAL_UNCERTAINTY_ASSIGNED_CONTEXT((#5496))
GLOBAL_UNIT_ASSIGNED_CONTEXT((#5506,#5508,#5509))
REPRESENTATION_CONTEXT('','3D')
);
#5506=(
LENGTH_UNIT()
NAMED_UNIT(*)
SI_UNIT(.MILLI.,.METRE.)
);
#5508=(
NAMED_UNIT(*)
PLANE_ANGLE_UNIT()
SI_UNIT($,.RADIAN.)
);
#5509=(
NAMED_UNIT(*)
SI_UNIT($,.STERADIAN.)
SOLID_ANGLE_UNIT()
);
#5511=SHAPE_DEFINITION_REPRESENTATION(#5519,#5537);
#5519=PRODUCT_DEFINITION_SHAPE('',$,#5546);
#5537=SHAPE_REPRESENTATION('',(#3379),#5498);
#5544=PRODUCT_DEFINITION_CONTEXT('part definition',#5570,'design');
#5546=PRODUCT_DEFINITION('Mast-bottom','Mast-bottom',#5554,#5544);
#5554=PRODUCT_DEFINITION_FORMATION('',$,#5573);
#5570=APPLICATION_CONTEXT(
'Core Data for Automotive Mechanical Design Process');
#5571=PRODUCT_CONTEXT('part definition',#5570,'mechanical');
#5573=PRODUCT('Mast-bottom','Mast-bottom','40x40x3mm-2pcs-mast-bottom',
(#5571));
#5581=PRESENTATION_STYLE_ASSIGNMENT((#5589));
#5589=SURFACE_STYLE_USAGE(.BOTH.,#5597);
#5597=SURFACE_SIDE_STYLE('',(#5605));
#5605=SURFACE_STYLE_FILL_AREA(#5613);
#5613=FILL_AREA_STYLE('Opaque(234,234,234)',(#5621));
#5621=FILL_AREA_STYLE_COLOUR('Opaque(234,234,234)',#5629);
#5629=COLOUR_RGB('Opaque(234,234,234)', 0.09019608, 0.27058824, 0.51372549);
ENDSEC;
END-ISO-10303-21;
